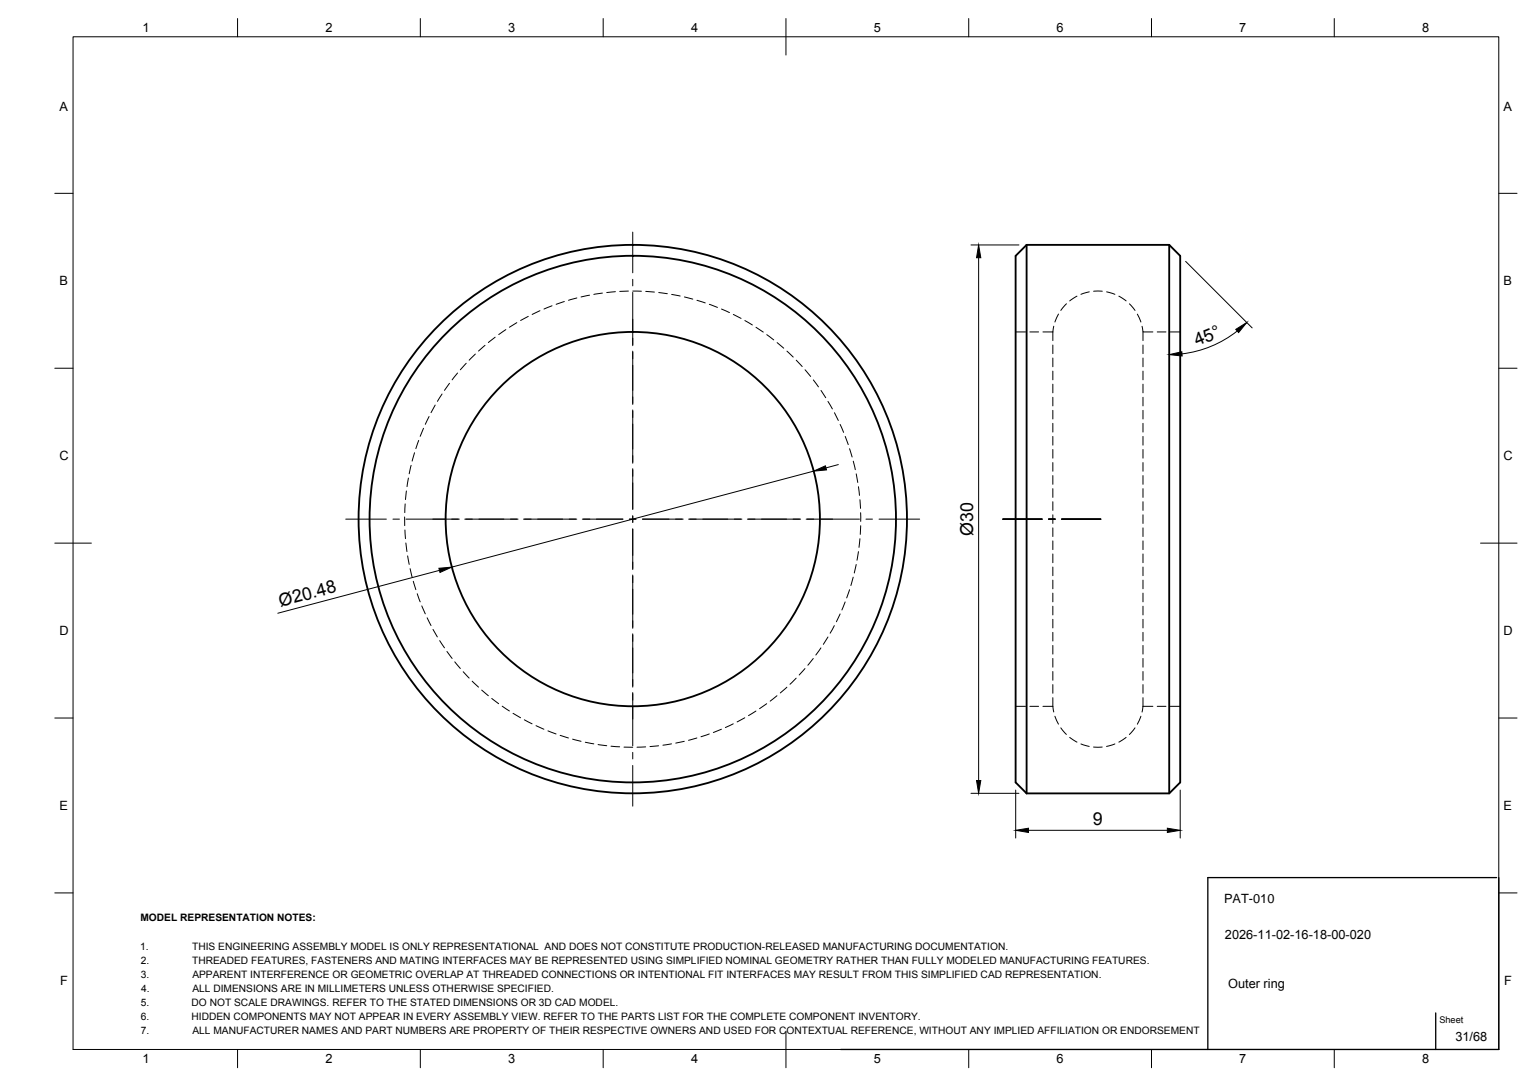
ISO-10303-21;
HEADER;
/* Generated by software containing ST-Developer
 * from STEP Tools, Inc. (www.steptools.com) 
 */

FILE_DESCRIPTION(
/* description */ ('Belt conveyor head drive unit'),
/* implementation_level */ '2;1');

FILE_NAME(
/* name */ 'Outer ring.step',
/* time_stamp */ '2026-10-28T03:26:19-07:00',
/* author */ (''),
/* organization */ (''),
/* preprocessor_version */ 'ST-DEVELOPER v20.2',
/* originating_system */ 'Autodesk Translation Framework v15.17.0.0',
/* authorisation */ '');

FILE_SCHEMA (('AUTOMOTIVE_DESIGN { 1 0 10303 214 3 1 1 }'));
ENDSEC;

DATA;
#10=MECHANICAL_DESIGN_GEOMETRIC_PRESENTATION_REPRESENTATION('',(#875),#27069);
#679=CONICAL_SURFACE('',#15222,1.47,0.785398163397449);
#680=CONICAL_SURFACE('',#15226,1.47,0.785398163397449);
#706=TOROIDAL_SURFACE('',#15211,1.,0.247676);
#737=SHAPE_REPRESENTATION_RELATIONSHIP('SRR','None',#27382,#806);
#806=ADVANCED_BREP_SHAPE_REPRESENTATION('',(#960),#27024);
#875=STYLED_ITEM('',(#27797),#960);
#960=MANIFOLD_SOLID_BREP('Body1',#13740);
#1153=FACE_BOUND('',#2887,.T.);
#1154=FACE_BOUND('',#2892,.T.);
#1439=PLANE('',#15219);
#1440=PLANE('',#15228);
#1943=FACE_OUTER_BOUND('',#2884,.T.);
#1944=FACE_OUTER_BOUND('',#2885,.T.);
#1945=FACE_OUTER_BOUND('',#2886,.T.);
#1946=FACE_OUTER_BOUND('',#2888,.T.);
#1947=FACE_OUTER_BOUND('',#2889,.T.);
#1948=FACE_OUTER_BOUND('',#2890,.T.);
#1949=FACE_OUTER_BOUND('',#2891,.T.);
#1950=FACE_OUTER_BOUND('',#2893,.T.);
#2884=EDGE_LOOP('',(#10304,#10305,#10306,#10307,#10308,#10309));
#2885=EDGE_LOOP('',(#10310,#10311,#10312,#10313,#10314));
#2886=EDGE_LOOP('',(#10315));
#2887=EDGE_LOOP('',(#10316));
#2888=EDGE_LOOP('',(#10317,#10318,#10319,#10320));
#2889=EDGE_LOOP('',(#10321,#10322,#10323,#10324));
#2890=EDGE_LOOP('',(#10325,#10326,#10327,#10328));
#2891=EDGE_LOOP('',(#10329));
#2892=EDGE_LOOP('',(#10330));
#2893=EDGE_LOOP('',(#10331,#10332,#10333,#10334,#10335));
#3864=LINE('',#22446,#4656);
#3865=LINE('',#22455,#4657);
#3866=LINE('',#22459,#4658);
#3867=LINE('',#22463,#4659);
#3868=LINE('',#22466,#4660);
#4656=VECTOR('',#18114,1.023815);
#4657=VECTOR('',#18125,1.47);
#4658=VECTOR('',#18130,1.5);
#4659=VECTOR('',#18135,1.47);
#4660=VECTOR('',#18140,1.023815);
#5389=CIRCLE('',#15212,1.023815);
#5390=CIRCLE('',#15213,1.023815);
#5391=CIRCLE('',#15214,0.247676);
#5392=CIRCLE('',#15215,1.023815);
#5393=CIRCLE('',#15216,1.023815);
#5394=CIRCLE('',#15218,1.023815);
#5395=CIRCLE('',#15220,1.44);
#5396=CIRCLE('',#15221,1.023815);
#5397=CIRCLE('',#15223,1.5);
#5398=CIRCLE('',#15225,1.5);
#5399=CIRCLE('',#15227,1.44);
#6401=VERTEX_POINT('',#22434);
#6402=VERTEX_POINT('',#22435);
#6403=VERTEX_POINT('',#22438);
#6404=VERTEX_POINT('',#22440);
#6405=VERTEX_POINT('',#22444);
#6406=VERTEX_POINT('',#22448);
#6407=VERTEX_POINT('',#22450);
#6408=VERTEX_POINT('',#22453);
#6409=VERTEX_POINT('',#22457);
#6410=VERTEX_POINT('',#22461);
#7844=EDGE_CURVE('',#6401,#6402,#5389,.T.);
#7845=EDGE_CURVE('',#6402,#6401,#5390,.T.);
#7846=EDGE_CURVE('',#6402,#6403,#5391,.T.);
#7847=EDGE_CURVE('',#6404,#6403,#5392,.T.);
#7848=EDGE_CURVE('',#6403,#6404,#5393,.T.);
#7849=EDGE_CURVE('',#6405,#6405,#5394,.T.);
#7850=EDGE_CURVE('',#6405,#6404,#3864,.T.);
#7851=EDGE_CURVE('',#6406,#6406,#5395,.T.);
#7852=EDGE_CURVE('',#6407,#6407,#5396,.T.);
#7853=EDGE_CURVE('',#6408,#6408,#5397,.T.);
#7854=EDGE_CURVE('',#6408,#6406,#3865,.T.);
#7855=EDGE_CURVE('',#6409,#6409,#5398,.T.);
#7856=EDGE_CURVE('',#6409,#6408,#3866,.T.);
#7857=EDGE_CURVE('',#6410,#6410,#5399,.T.);
#7858=EDGE_CURVE('',#6410,#6409,#3867,.T.);
#7859=EDGE_CURVE('',#6401,#6407,#3868,.T.);
#10304=ORIENTED_EDGE('',*,*,#7844,.F.);
#10305=ORIENTED_EDGE('',*,*,#7845,.F.);
#10306=ORIENTED_EDGE('',*,*,#7846,.T.);
#10307=ORIENTED_EDGE('',*,*,#7847,.F.);
#10308=ORIENTED_EDGE('',*,*,#7848,.F.);
#10309=ORIENTED_EDGE('',*,*,#7846,.F.);
#10310=ORIENTED_EDGE('',*,*,#7849,.T.);
#10311=ORIENTED_EDGE('',*,*,#7850,.T.);
#10312=ORIENTED_EDGE('',*,*,#7847,.T.);
#10313=ORIENTED_EDGE('',*,*,#7848,.T.);
#10314=ORIENTED_EDGE('',*,*,#7850,.F.);
#10315=ORIENTED_EDGE('',*,*,#7851,.F.);
#10316=ORIENTED_EDGE('',*,*,#7852,.T.);
#10317=ORIENTED_EDGE('',*,*,#7853,.F.);
#10318=ORIENTED_EDGE('',*,*,#7854,.T.);
#10319=ORIENTED_EDGE('',*,*,#7851,.T.);
#10320=ORIENTED_EDGE('',*,*,#7854,.F.);
#10321=ORIENTED_EDGE('',*,*,#7855,.F.);
#10322=ORIENTED_EDGE('',*,*,#7856,.T.);
#10323=ORIENTED_EDGE('',*,*,#7853,.T.);
#10324=ORIENTED_EDGE('',*,*,#7856,.F.);
#10325=ORIENTED_EDGE('',*,*,#7857,.F.);
#10326=ORIENTED_EDGE('',*,*,#7858,.T.);
#10327=ORIENTED_EDGE('',*,*,#7855,.T.);
#10328=ORIENTED_EDGE('',*,*,#7858,.F.);
#10329=ORIENTED_EDGE('',*,*,#7857,.T.);
#10330=ORIENTED_EDGE('',*,*,#7849,.F.);
#10331=ORIENTED_EDGE('',*,*,#7844,.T.);
#10332=ORIENTED_EDGE('',*,*,#7845,.T.);
#10333=ORIENTED_EDGE('',*,*,#7859,.T.);
#10334=ORIENTED_EDGE('',*,*,#7852,.F.);
#10335=ORIENTED_EDGE('',*,*,#7859,.F.);
#12677=CYLINDRICAL_SURFACE('',#15217,1.023815);
#12678=CYLINDRICAL_SURFACE('',#15224,1.5);
#12679=CYLINDRICAL_SURFACE('',#15229,1.023815);
#13222=ADVANCED_FACE('',(#1943),#706,.F.);
#13223=ADVANCED_FACE('',(#1944),#12677,.F.);
#13224=ADVANCED_FACE('',(#1945,#1153),#1439,.T.);
#13225=ADVANCED_FACE('',(#1946),#679,.T.);
#13226=ADVANCED_FACE('',(#1947),#12678,.T.);
#13227=ADVANCED_FACE('',(#1948),#680,.T.);
#13228=ADVANCED_FACE('',(#1949,#1154),#1440,.T.);
#13229=ADVANCED_FACE('',(#1950),#12679,.F.);
#13740=CLOSED_SHELL('',(#13222,#13223,#13224,#13225,#13226,#13227,#13228,
#13229));
#15210=AXIS2_PLACEMENT_3D('',#22432,#18096,#18097);
#15211=AXIS2_PLACEMENT_3D('',#22433,#18098,#18099);
#15212=AXIS2_PLACEMENT_3D('',#22436,#18100,#18101);
#15213=AXIS2_PLACEMENT_3D('',#22437,#18102,#18103);
#15214=AXIS2_PLACEMENT_3D('',#22439,#18104,#18105);
#15215=AXIS2_PLACEMENT_3D('',#22441,#18106,#18107);
#15216=AXIS2_PLACEMENT_3D('',#22442,#18108,#18109);
#15217=AXIS2_PLACEMENT_3D('',#22443,#18110,#18111);
#15218=AXIS2_PLACEMENT_3D('',#22445,#18112,#18113);
#15219=AXIS2_PLACEMENT_3D('',#22447,#18115,#18116);
#15220=AXIS2_PLACEMENT_3D('',#22449,#18117,#18118);
#15221=AXIS2_PLACEMENT_3D('',#22451,#18119,#18120);
#15222=AXIS2_PLACEMENT_3D('',#22452,#18121,#18122);
#15223=AXIS2_PLACEMENT_3D('',#22454,#18123,#18124);
#15224=AXIS2_PLACEMENT_3D('',#22456,#18126,#18127);
#15225=AXIS2_PLACEMENT_3D('',#22458,#18128,#18129);
#15226=AXIS2_PLACEMENT_3D('',#22460,#18131,#18132);
#15227=AXIS2_PLACEMENT_3D('',#22462,#18133,#18134);
#15228=AXIS2_PLACEMENT_3D('',#22464,#18136,#18137);
#15229=AXIS2_PLACEMENT_3D('',#22465,#18138,#18139);
#18096=DIRECTION('axis',(0.,0.,1.));
#18097=DIRECTION('refdir',(1.,0.,0.));
#18098=DIRECTION('center_axis',(0.,-1.,0.));
#18099=DIRECTION('ref_axis',(0.,0.,-1.));
#18100=DIRECTION('center_axis',(0.,-1.,0.));
#18101=DIRECTION('ref_axis',(1.,0.,0.));
#18102=DIRECTION('center_axis',(0.,-1.,0.));
#18103=DIRECTION('ref_axis',(1.,0.,0.));
#18104=DIRECTION('center_axis',(1.,0.,1.22464679914735E-16));
#18105=DIRECTION('ref_axis',(-1.22464679914735E-16,0.,1.));
#18106=DIRECTION('center_axis',(0.,1.,0.));
#18107=DIRECTION('ref_axis',(1.,0.,0.));
#18108=DIRECTION('center_axis',(0.,1.,0.));
#18109=DIRECTION('ref_axis',(1.,0.,0.));
#18110=DIRECTION('center_axis',(0.,-1.,0.));
#18111=DIRECTION('ref_axis',(1.,0.,0.));
#18112=DIRECTION('center_axis',(0.,-1.,0.));
#18113=DIRECTION('ref_axis',(1.,0.,0.));
#18114=DIRECTION('',(0.,1.,0.));
#18115=DIRECTION('center_axis',(0.,1.,0.));
#18116=DIRECTION('ref_axis',(0.,0.,1.));
#18117=DIRECTION('center_axis',(0.,-1.,0.));
#18118=DIRECTION('ref_axis',(1.,0.,0.));
#18119=DIRECTION('center_axis',(0.,-1.,0.));
#18120=DIRECTION('ref_axis',(1.,0.,0.));
#18121=DIRECTION('center_axis',(0.,-1.,0.));
#18122=DIRECTION('ref_axis',(1.,0.,0.));
#18123=DIRECTION('center_axis',(0.,-1.,0.));
#18124=DIRECTION('ref_axis',(1.,0.,0.));
#18125=DIRECTION('',(0.707106781186548,0.707106781186547,8.65956056235494E-17));
#18126=DIRECTION('center_axis',(0.,-1.,0.));
#18127=DIRECTION('ref_axis',(1.,0.,0.));
#18128=DIRECTION('center_axis',(0.,-1.,0.));
#18129=DIRECTION('ref_axis',(1.,0.,0.));
#18130=DIRECTION('',(0.,1.,0.));
#18131=DIRECTION('center_axis',(0.,1.,0.));
#18132=DIRECTION('ref_axis',(1.,0.,0.));
#18133=DIRECTION('center_axis',(0.,-1.,0.));
#18134=DIRECTION('ref_axis',(1.,0.,0.));
#18135=DIRECTION('',(-0.707106781186548,0.707106781186547,-8.65956056235494E-17));
#18136=DIRECTION('center_axis',(0.,-1.,0.));
#18137=DIRECTION('ref_axis',(0.,0.,-1.));
#18138=DIRECTION('center_axis',(0.,-1.,0.));
#18139=DIRECTION('ref_axis',(1.,0.,0.));
#18140=DIRECTION('',(0.,1.,0.));
#22432=CARTESIAN_POINT('',(0.,0.,0.));
#22433=CARTESIAN_POINT('Origin',(0.,0.,0.));
#22434=CARTESIAN_POINT('',(-1.023815,0.246528389340863,-1.25381176266905E-16));
#22435=CARTESIAN_POINT('',(-1.25381176266905E-16,0.246528389340863,1.023815));
#22436=CARTESIAN_POINT('Origin',(0.,0.246528389340863,0.));
#22437=CARTESIAN_POINT('Origin',(0.,0.246528389340863,0.));
#22438=CARTESIAN_POINT('',(-1.25381176266905E-16,-0.246528389340863,1.023815));
#22439=CARTESIAN_POINT('Origin',(-1.22464679914735E-16,0.,1.));
#22440=CARTESIAN_POINT('',(-1.023815,-0.246528389340863,1.25381176266905E-16));
#22441=CARTESIAN_POINT('Origin',(0.,-0.246528389340863,0.));
#22442=CARTESIAN_POINT('Origin',(0.,-0.246528389340863,0.));
#22443=CARTESIAN_POINT('Origin',(0.,0.,0.));
#22444=CARTESIAN_POINT('',(-1.023815,-0.45,-1.25381176266905E-16));
#22445=CARTESIAN_POINT('Origin',(0.,-0.45,0.));
#22446=CARTESIAN_POINT('',(-1.023815,0.,-1.25381176266905E-16));
#22447=CARTESIAN_POINT('Origin',(1.44,0.45,0.));
#22448=CARTESIAN_POINT('',(-1.44,0.45,-1.76349139077219E-16));
#22449=CARTESIAN_POINT('Origin',(0.,0.45,0.));
#22450=CARTESIAN_POINT('',(-1.023815,0.45,-1.25381176266905E-16));
#22451=CARTESIAN_POINT('Origin',(0.,0.45,0.));
#22452=CARTESIAN_POINT('Origin',(0.,0.42,0.));
#22453=CARTESIAN_POINT('',(-1.5,0.39,-1.83697019872103E-16));
#22454=CARTESIAN_POINT('Origin',(0.,0.39,0.));
#22455=CARTESIAN_POINT('',(-1.47,0.42,-1.80023079474661E-16));
#22456=CARTESIAN_POINT('Origin',(0.,0.,0.));
#22457=CARTESIAN_POINT('',(-1.5,-0.39,-1.83697019872103E-16));
#22458=CARTESIAN_POINT('Origin',(0.,-0.39,0.));
#22459=CARTESIAN_POINT('',(-1.5,0.,-1.83697019872103E-16));
#22460=CARTESIAN_POINT('Origin',(0.,-0.42,0.));
#22461=CARTESIAN_POINT('',(-1.44,-0.45,-1.76349139077219E-16));
#22462=CARTESIAN_POINT('Origin',(0.,-0.45,0.));
#22463=CARTESIAN_POINT('',(-1.47,-0.42,-1.80023079474661E-16));
#22464=CARTESIAN_POINT('Origin',(1.023815,-0.45,0.));
#22465=CARTESIAN_POINT('Origin',(0.,0.,0.));
#22466=CARTESIAN_POINT('',(-1.023815,0.,-1.25381176266905E-16));
#26947=UNCERTAINTY_MEASURE_WITH_UNIT(LENGTH_MEASURE(0.001),#27070,
'DISTANCE_ACCURACY_VALUE',
'Maximum model space distance between geometric entities at asserted c
onnectivities');
#26992=UNCERTAINTY_MEASURE_WITH_UNIT(LENGTH_MEASURE(0.001),#27070,
'DISTANCE_ACCURACY_VALUE',
'Maximum model space distance between geometric entities at asserted c
onnectivities');
#27024=(
GEOMETRIC_REPRESENTATION_CONTEXT(3)
GLOBAL_UNCERTAINTY_ASSIGNED_CONTEXT((#26947))
GLOBAL_UNIT_ASSIGNED_CONTEXT((#27070,#27072,#27073))
REPRESENTATION_CONTEXT('','3D')
);
#27069=(
GEOMETRIC_REPRESENTATION_CONTEXT(3)
GLOBAL_UNCERTAINTY_ASSIGNED_CONTEXT((#26992))
GLOBAL_UNIT_ASSIGNED_CONTEXT((#27070,#27072,#27073))
REPRESENTATION_CONTEXT('','3D')
);
#27070=(
LENGTH_UNIT()
NAMED_UNIT(*)
SI_UNIT(.CENTI.,.METRE.)
);
#27072=(
NAMED_UNIT(*)
PLANE_ANGLE_UNIT()
SI_UNIT($,.RADIAN.)
);
#27073=(
NAMED_UNIT(*)
SI_UNIT($,.STERADIAN.)
SOLID_ANGLE_UNIT()
);
#27105=SHAPE_DEFINITION_REPRESENTATION(#27181,#27382);
#27181=PRODUCT_DEFINITION_SHAPE('',$,#27459);
#27382=SHAPE_REPRESENTATION('',(#15210),#27024);
#27427=PRODUCT_DEFINITION_CONTEXT('part definition',#27657,'design');
#27459=PRODUCT_DEFINITION('Outer ring','Outer ring',#27535,#27427);
#27535=PRODUCT_DEFINITION_FORMATION('',$,#27690);
#27657=APPLICATION_CONTEXT(
'Core Data for Automotive Mechanical Design Process');
#27658=PRODUCT_CONTEXT('part definition',#27657,'mechanical');
#27690=PRODUCT('Outer ring','Outer ring','Outer ring',(#27658));
#27791=COLOUR_RGB('Grey',0.48,0.52,0.57);
#27792=FILL_AREA_STYLE_COLOUR('',#27791);
#27793=FILL_AREA_STYLE('',(#27792));
#27794=SURFACE_STYLE_FILL_AREA(#27793);
#27795=SURFACE_SIDE_STYLE('',(#27794));
#27796=SURFACE_STYLE_USAGE(.BOTH.,#27795);
#27797=PRESENTATION_STYLE_ASSIGNMENT((#27796));
ENDSEC;
END-ISO-10303-21;
